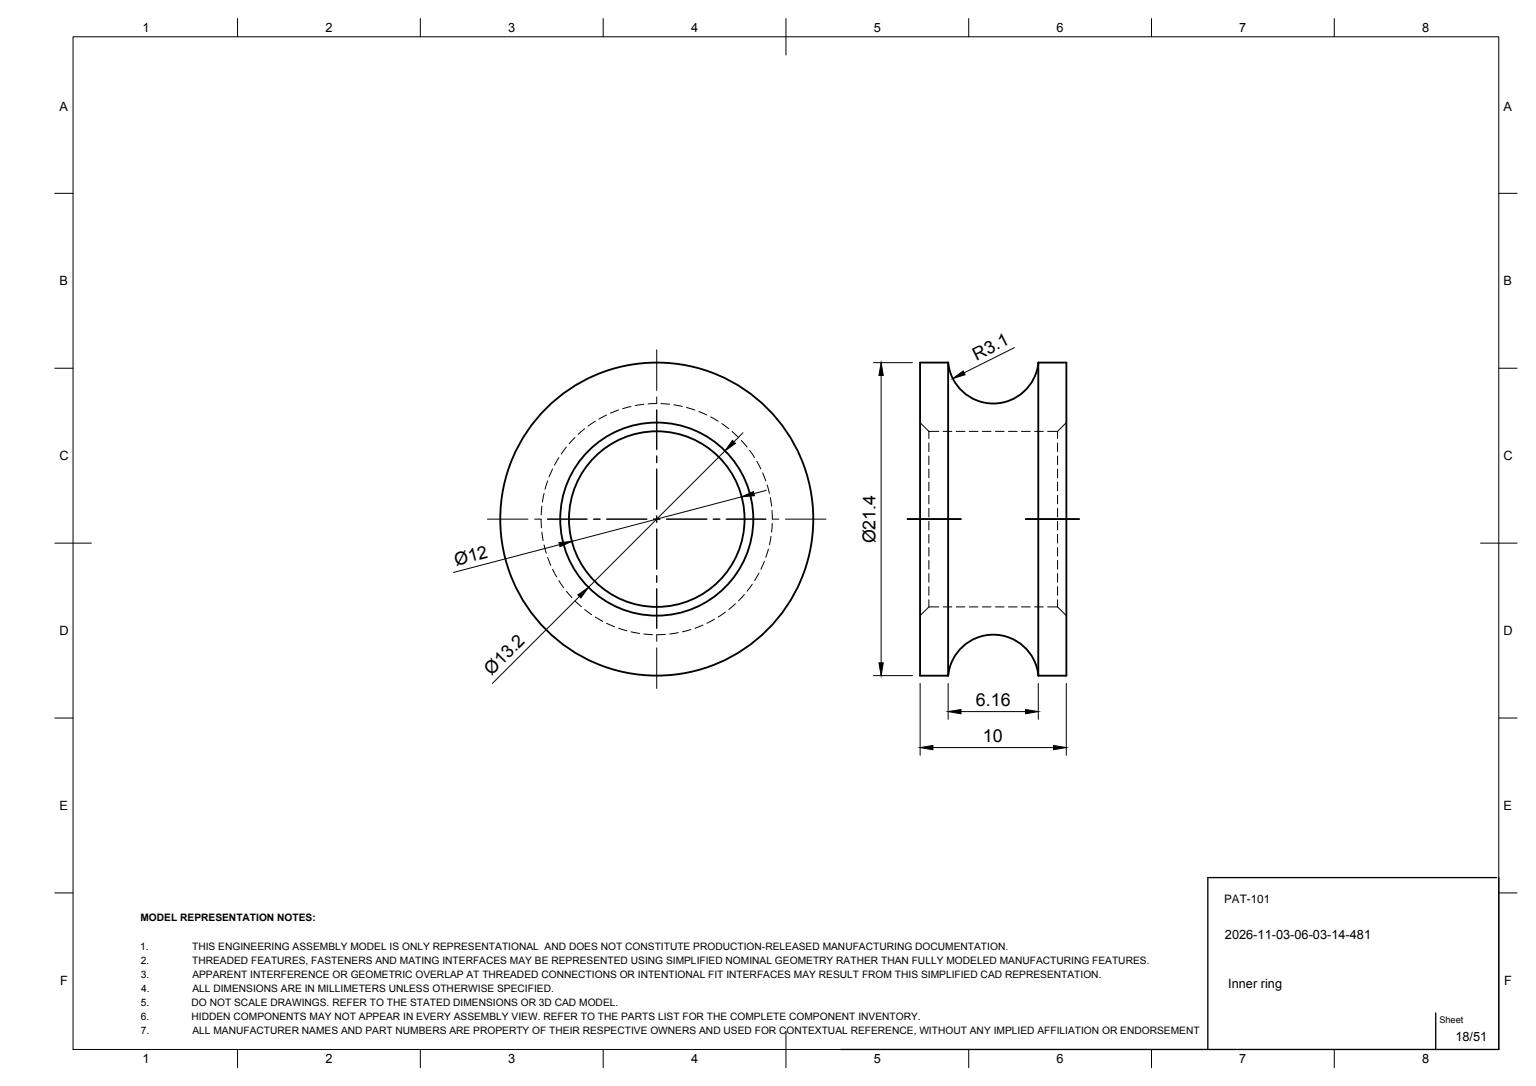
ISO-10303-21;
HEADER;
/* Generated by software containing ST-Developer
 * from STEP Tools, Inc. (www.steptools.com) 
 */

FILE_DESCRIPTION(
/* description */ ('Spur gear reduction stage 2-1 on bearing plates'),
/* implementation_level */ '2;1');

FILE_NAME(
/* name */ 'Inner ring.step',
/* time_stamp */ '2026-10-28T03:22:07-07:00',
/* author */ (''),
/* organization */ (''),
/* preprocessor_version */ 'ST-DEVELOPER v20.2',
/* originating_system */ 'Autodesk Translation Framework v15.17.0.0',
/* authorisation */ '');

FILE_SCHEMA (('AUTOMOTIVE_DESIGN { 1 0 10303 214 3 1 1 }'));
ENDSEC;

DATA;
#10=MECHANICAL_DESIGN_GEOMETRIC_PRESENTATION_REPRESENTATION('',(#960),#53909);
#825=TOROIDAL_SURFACE('',#12155,1.1,0.309556);
#840=CONICAL_SURFACE('',#12166,0.63,0.785398163397448);
#841=CONICAL_SURFACE('',#12173,0.63,0.785398163397448);
#874=SHAPE_REPRESENTATION_RELATIONSHIP('SRR','None',#54102,#917);
#917=ADVANCED_BREP_SHAPE_REPRESENTATION('',(#1016),#53876);
#960=STYLED_ITEM('',(#54397),#1016);
#1016=MANIFOLD_SOLID_BREP('Body1',#11286);
#1178=FACE_BOUND('',#2438,.T.);
#1179=FACE_BOUND('',#2441,.T.);
#1314=PLANE('',#12168);
#1315=PLANE('',#12171);
#1667=FACE_OUTER_BOUND('',#2433,.T.);
#1668=FACE_OUTER_BOUND('',#2434,.T.);
#1669=FACE_OUTER_BOUND('',#2435,.T.);
#1670=FACE_OUTER_BOUND('',#2436,.T.);
#1671=FACE_OUTER_BOUND('',#2437,.T.);
#1672=FACE_OUTER_BOUND('',#2439,.T.);
#1673=FACE_OUTER_BOUND('',#2440,.T.);
#1674=FACE_OUTER_BOUND('',#2442,.T.);
#2433=EDGE_LOOP('',(#8008,#8009,#8010,#8011,#8012,#8013));
#2434=EDGE_LOOP('',(#8014,#8015,#8016,#8017,#8018));
#2435=EDGE_LOOP('',(#8019,#8020,#8021,#8022));
#2436=EDGE_LOOP('',(#8023,#8024,#8025,#8026));
#2437=EDGE_LOOP('',(#8027));
#2438=EDGE_LOOP('',(#8028));
#2439=EDGE_LOOP('',(#8029,#8030,#8031,#8032,#8033));
#2440=EDGE_LOOP('',(#8034));
#2441=EDGE_LOOP('',(#8035));
#2442=EDGE_LOOP('',(#8036,#8037,#8038,#8039));
#3137=LINE('',#16712,#3778);
#3138=LINE('',#16718,#3779);
#3139=LINE('',#16722,#3780);
#3140=LINE('',#16728,#3781);
#3141=LINE('',#16733,#3782);
#3778=VECTOR('',#13854,1.070235);
#3779=VECTOR('',#13861,0.6);
#3780=VECTOR('',#13866,0.63);
#3781=VECTOR('',#13875,1.070235);
#3782=VECTOR('',#13882,0.63);
#4427=CIRCLE('',#12156,1.070235);
#4428=CIRCLE('',#12157,1.070235);
#4429=CIRCLE('',#12158,0.309556);
#4430=CIRCLE('',#12159,1.070235);
#4431=CIRCLE('',#12160,1.070235);
#4432=CIRCLE('',#12162,1.070235);
#4433=CIRCLE('',#12164,0.6);
#4434=CIRCLE('',#12165,0.6);
#4435=CIRCLE('',#12167,0.66);
#4436=CIRCLE('',#12170,1.070235);
#4437=CIRCLE('',#12172,0.66);
#5000=VERTEX_POINT('',#16701);
#5001=VERTEX_POINT('',#16702);
#5002=VERTEX_POINT('',#16705);
#5003=VERTEX_POINT('',#16707);
#5004=VERTEX_POINT('',#16711);
#5005=VERTEX_POINT('',#16715);
#5006=VERTEX_POINT('',#16717);
#5007=VERTEX_POINT('',#16721);
#5008=VERTEX_POINT('',#16726);
#5009=VERTEX_POINT('',#16730);
#6146=EDGE_CURVE('',#5000,#5001,#4427,.T.);
#6147=EDGE_CURVE('',#5001,#5000,#4428,.T.);
#6148=EDGE_CURVE('',#5001,#5002,#4429,.T.);
#6149=EDGE_CURVE('',#5003,#5002,#4430,.T.);
#6150=EDGE_CURVE('',#5002,#5003,#4431,.T.);
#6151=EDGE_CURVE('',#5003,#5004,#3137,.T.);
#6152=EDGE_CURVE('',#5004,#5004,#4432,.T.);
#6153=EDGE_CURVE('',#5005,#5005,#4433,.T.);
#6154=EDGE_CURVE('',#5005,#5006,#3138,.T.);
#6155=EDGE_CURVE('',#5006,#5006,#4434,.T.);
#6156=EDGE_CURVE('',#5006,#5007,#3139,.T.);
#6157=EDGE_CURVE('',#5007,#5007,#4435,.T.);
#6158=EDGE_CURVE('',#5008,#5008,#4436,.T.);
#6159=EDGE_CURVE('',#5008,#5000,#3140,.T.);
#6160=EDGE_CURVE('',#5009,#5009,#4437,.T.);
#6161=EDGE_CURVE('',#5009,#5005,#3141,.T.);
#8008=ORIENTED_EDGE('',*,*,#6146,.F.);
#8009=ORIENTED_EDGE('',*,*,#6147,.F.);
#8010=ORIENTED_EDGE('',*,*,#6148,.T.);
#8011=ORIENTED_EDGE('',*,*,#6149,.F.);
#8012=ORIENTED_EDGE('',*,*,#6150,.F.);
#8013=ORIENTED_EDGE('',*,*,#6148,.F.);
#8014=ORIENTED_EDGE('',*,*,#6149,.T.);
#8015=ORIENTED_EDGE('',*,*,#6150,.T.);
#8016=ORIENTED_EDGE('',*,*,#6151,.T.);
#8017=ORIENTED_EDGE('',*,*,#6152,.T.);
#8018=ORIENTED_EDGE('',*,*,#6151,.F.);
#8019=ORIENTED_EDGE('',*,*,#6153,.T.);
#8020=ORIENTED_EDGE('',*,*,#6154,.T.);
#8021=ORIENTED_EDGE('',*,*,#6155,.F.);
#8022=ORIENTED_EDGE('',*,*,#6154,.F.);
#8023=ORIENTED_EDGE('',*,*,#6155,.T.);
#8024=ORIENTED_EDGE('',*,*,#6156,.T.);
#8025=ORIENTED_EDGE('',*,*,#6157,.F.);
#8026=ORIENTED_EDGE('',*,*,#6156,.F.);
#8027=ORIENTED_EDGE('',*,*,#6152,.F.);
#8028=ORIENTED_EDGE('',*,*,#6157,.T.);
#8029=ORIENTED_EDGE('',*,*,#6158,.F.);
#8030=ORIENTED_EDGE('',*,*,#6159,.T.);
#8031=ORIENTED_EDGE('',*,*,#6146,.T.);
#8032=ORIENTED_EDGE('',*,*,#6147,.T.);
#8033=ORIENTED_EDGE('',*,*,#6159,.F.);
#8034=ORIENTED_EDGE('',*,*,#6158,.T.);
#8035=ORIENTED_EDGE('',*,*,#6160,.F.);
#8036=ORIENTED_EDGE('',*,*,#6160,.T.);
#8037=ORIENTED_EDGE('',*,*,#6161,.T.);
#8038=ORIENTED_EDGE('',*,*,#6153,.F.);
#8039=ORIENTED_EDGE('',*,*,#6161,.F.);
#10500=CYLINDRICAL_SURFACE('',#12161,1.070235);
#10501=CYLINDRICAL_SURFACE('',#12163,0.6);
#10502=CYLINDRICAL_SURFACE('',#12169,1.070235);
#10787=ADVANCED_FACE('',(#1667),#825,.F.);
#10788=ADVANCED_FACE('',(#1668),#10500,.T.);
#10789=ADVANCED_FACE('',(#1669),#10501,.F.);
#10790=ADVANCED_FACE('',(#1670),#840,.F.);
#10791=ADVANCED_FACE('',(#1671,#1178),#1314,.T.);
#10792=ADVANCED_FACE('',(#1672),#10502,.T.);
#10793=ADVANCED_FACE('',(#1673,#1179),#1315,.T.);
#10794=ADVANCED_FACE('',(#1674),#841,.F.);
#11286=CLOSED_SHELL('',(#10787,#10788,#10789,#10790,#10791,#10792,#10793,
#10794));
#12154=AXIS2_PLACEMENT_3D('',#16699,#13838,#13839);
#12155=AXIS2_PLACEMENT_3D('',#16700,#13840,#13841);
#12156=AXIS2_PLACEMENT_3D('',#16703,#13842,#13843);
#12157=AXIS2_PLACEMENT_3D('',#16704,#13844,#13845);
#12158=AXIS2_PLACEMENT_3D('',#16706,#13846,#13847);
#12159=AXIS2_PLACEMENT_3D('',#16708,#13848,#13849);
#12160=AXIS2_PLACEMENT_3D('',#16709,#13850,#13851);
#12161=AXIS2_PLACEMENT_3D('',#16710,#13852,#13853);
#12162=AXIS2_PLACEMENT_3D('',#16713,#13855,#13856);
#12163=AXIS2_PLACEMENT_3D('',#16714,#13857,#13858);
#12164=AXIS2_PLACEMENT_3D('',#16716,#13859,#13860);
#12165=AXIS2_PLACEMENT_3D('',#16719,#13862,#13863);
#12166=AXIS2_PLACEMENT_3D('',#16720,#13864,#13865);
#12167=AXIS2_PLACEMENT_3D('',#16723,#13867,#13868);
#12168=AXIS2_PLACEMENT_3D('',#16724,#13869,#13870);
#12169=AXIS2_PLACEMENT_3D('',#16725,#13871,#13872);
#12170=AXIS2_PLACEMENT_3D('',#16727,#13873,#13874);
#12171=AXIS2_PLACEMENT_3D('',#16729,#13876,#13877);
#12172=AXIS2_PLACEMENT_3D('',#16731,#13878,#13879);
#12173=AXIS2_PLACEMENT_3D('',#16732,#13880,#13881);
#13838=DIRECTION('axis',(0.,0.,1.));
#13839=DIRECTION('refdir',(1.,0.,0.));
#13840=DIRECTION('center_axis',(0.,-1.,0.));
#13841=DIRECTION('ref_axis',(0.,0.,-1.));
#13842=DIRECTION('center_axis',(0.,-1.,0.));
#13843=DIRECTION('ref_axis',(1.,0.,0.));
#13844=DIRECTION('center_axis',(0.,-1.,0.));
#13845=DIRECTION('ref_axis',(1.,0.,0.));
#13846=DIRECTION('center_axis',(1.,0.,1.22464679914735E-16));
#13847=DIRECTION('ref_axis',(-1.22464679914735E-16,0.,1.));
#13848=DIRECTION('center_axis',(0.,1.,0.));
#13849=DIRECTION('ref_axis',(1.,0.,0.));
#13850=DIRECTION('center_axis',(0.,1.,0.));
#13851=DIRECTION('ref_axis',(1.,0.,0.));
#13852=DIRECTION('center_axis',(0.,-1.,0.));
#13853=DIRECTION('ref_axis',(1.,0.,0.));
#13854=DIRECTION('',(0.,1.,0.));
#13855=DIRECTION('center_axis',(0.,-1.,0.));
#13856=DIRECTION('ref_axis',(1.,0.,0.));
#13857=DIRECTION('center_axis',(0.,-1.,0.));
#13858=DIRECTION('ref_axis',(1.,0.,0.));
#13859=DIRECTION('center_axis',(0.,-1.,0.));
#13860=DIRECTION('ref_axis',(1.,0.,0.));
#13861=DIRECTION('',(0.,1.,0.));
#13862=DIRECTION('center_axis',(0.,-1.,0.));
#13863=DIRECTION('ref_axis',(1.,0.,0.));
#13864=DIRECTION('center_axis',(0.,1.,0.));
#13865=DIRECTION('ref_axis',(1.,0.,0.));
#13866=DIRECTION('',(-0.707106781186548,0.707106781186547,-8.65956056235493E-17));
#13867=DIRECTION('center_axis',(0.,-1.,0.));
#13868=DIRECTION('ref_axis',(1.,0.,0.));
#13869=DIRECTION('center_axis',(0.,1.,0.));
#13870=DIRECTION('ref_axis',(0.,0.,1.));
#13871=DIRECTION('center_axis',(0.,-1.,0.));
#13872=DIRECTION('ref_axis',(1.,0.,0.));
#13873=DIRECTION('center_axis',(0.,-1.,0.));
#13874=DIRECTION('ref_axis',(1.,0.,0.));
#13875=DIRECTION('',(0.,1.,0.));
#13876=DIRECTION('center_axis',(0.,-1.,0.));
#13877=DIRECTION('ref_axis',(0.,0.,-1.));
#13878=DIRECTION('center_axis',(0.,-1.,0.));
#13879=DIRECTION('ref_axis',(1.,0.,0.));
#13880=DIRECTION('center_axis',(0.,-1.,0.));
#13881=DIRECTION('ref_axis',(1.,0.,0.));
#13882=DIRECTION('',(0.707106781186548,0.707106781186547,8.65956056235493E-17));
#16699=CARTESIAN_POINT('',(0.,0.,0.));
#16700=CARTESIAN_POINT('Origin',(0.,0.,0.));
#16701=CARTESIAN_POINT('',(-1.070235,-0.308121667383195,-1.31065986708547E-16));
#16702=CARTESIAN_POINT('',(-1.31065986708547E-16,-0.308121667383195,1.070235));
#16703=CARTESIAN_POINT('Origin',(0.,-0.308121667383195,0.));
#16704=CARTESIAN_POINT('Origin',(0.,-0.308121667383195,0.));
#16705=CARTESIAN_POINT('',(-1.31065986708547E-16,0.308121667383195,1.070235));
#16706=CARTESIAN_POINT('Origin',(-1.34711147906209E-16,0.,1.1));
#16707=CARTESIAN_POINT('',(-1.070235,0.308121667383195,1.31065986708547E-16));
#16708=CARTESIAN_POINT('Origin',(0.,0.308121667383195,0.));
#16709=CARTESIAN_POINT('Origin',(0.,0.308121667383195,0.));
#16710=CARTESIAN_POINT('Origin',(0.,0.,0.));
#16711=CARTESIAN_POINT('',(-1.070235,0.5,-1.31065986708547E-16));
#16712=CARTESIAN_POINT('',(-1.070235,0.,-1.31065986708547E-16));
#16713=CARTESIAN_POINT('Origin',(0.,0.5,0.));
#16714=CARTESIAN_POINT('Origin',(0.,0.,0.));
#16715=CARTESIAN_POINT('',(-0.6,-0.44,-7.34788079488412E-17));
#16716=CARTESIAN_POINT('Origin',(0.,-0.44,0.));
#16717=CARTESIAN_POINT('',(-0.6,0.44,-7.34788079488412E-17));
#16718=CARTESIAN_POINT('',(-0.6,0.,-7.34788079488412E-17));
#16719=CARTESIAN_POINT('Origin',(0.,0.44,0.));
#16720=CARTESIAN_POINT('Origin',(0.,0.47,0.));
#16721=CARTESIAN_POINT('',(-0.66,0.5,-8.08266887437253E-17));
#16722=CARTESIAN_POINT('',(-0.63,0.47,-7.71527483462832E-17));
#16723=CARTESIAN_POINT('Origin',(0.,0.5,0.));
#16724=CARTESIAN_POINT('Origin',(1.070235,0.5,0.));
#16725=CARTESIAN_POINT('Origin',(0.,0.,0.));
#16726=CARTESIAN_POINT('',(-1.070235,-0.5,-1.31065986708547E-16));
#16727=CARTESIAN_POINT('Origin',(0.,-0.5,0.));
#16728=CARTESIAN_POINT('',(-1.070235,0.,-1.31065986708547E-16));
#16729=CARTESIAN_POINT('Origin',(0.66,-0.5,0.));
#16730=CARTESIAN_POINT('',(-0.66,-0.5,-8.08266887437253E-17));
#16731=CARTESIAN_POINT('Origin',(0.,-0.5,0.));
#16732=CARTESIAN_POINT('Origin',(0.,-0.47,0.));
#16733=CARTESIAN_POINT('',(-0.63,-0.47,-7.71527483462832E-17));
#53826=UNCERTAINTY_MEASURE_WITH_UNIT(LENGTH_MEASURE(0.001),#53910,
'DISTANCE_ACCURACY_VALUE',
'Maximum model space distance between geometric entities at asserted c
onnectivities');
#53859=UNCERTAINTY_MEASURE_WITH_UNIT(LENGTH_MEASURE(0.001),#53910,
'DISTANCE_ACCURACY_VALUE',
'Maximum model space distance between geometric entities at asserted c
onnectivities');
#53876=(
GEOMETRIC_REPRESENTATION_CONTEXT(3)
GLOBAL_UNCERTAINTY_ASSIGNED_CONTEXT((#53826))
GLOBAL_UNIT_ASSIGNED_CONTEXT((#53910,#53912,#53913))
REPRESENTATION_CONTEXT('','3D')
);
#53909=(
GEOMETRIC_REPRESENTATION_CONTEXT(3)
GLOBAL_UNCERTAINTY_ASSIGNED_CONTEXT((#53859))
GLOBAL_UNIT_ASSIGNED_CONTEXT((#53910,#53912,#53913))
REPRESENTATION_CONTEXT('','3D')
);
#53910=(
LENGTH_UNIT()
NAMED_UNIT(*)
SI_UNIT(.CENTI.,.METRE.)
);
#53912=(
NAMED_UNIT(*)
PLANE_ANGLE_UNIT()
SI_UNIT($,.RADIAN.)
);
#53913=(
NAMED_UNIT(*)
SI_UNIT($,.STERADIAN.)
SOLID_ANGLE_UNIT()
);
#53930=SHAPE_DEFINITION_REPRESENTATION(#53979,#54102);
#53979=PRODUCT_DEFINITION_SHAPE('',$,#54152);
#54102=SHAPE_REPRESENTATION('',(#12154),#53876);
#54135=PRODUCT_DEFINITION_CONTEXT('part definition',#54284,'design');
#54152=PRODUCT_DEFINITION('Inner ring','Inner ring',#54201,#54135);
#54201=PRODUCT_DEFINITION_FORMATION('',$,#54302);
#54284=APPLICATION_CONTEXT(
'Core Data for Automotive Mechanical Design Process');
#54285=PRODUCT_CONTEXT('part definition',#54284,'mechanical');
#54302=PRODUCT('Inner ring','Inner ring','Inner ring',(#54285));
#54391=COLOUR_RGB('Grey',0.48,0.52,0.57);
#54392=FILL_AREA_STYLE_COLOUR('',#54391);
#54393=FILL_AREA_STYLE('',(#54392));
#54394=SURFACE_STYLE_FILL_AREA(#54393);
#54395=SURFACE_SIDE_STYLE('',(#54394));
#54396=SURFACE_STYLE_USAGE(.BOTH.,#54395);
#54397=PRESENTATION_STYLE_ASSIGNMENT((#54396));
ENDSEC;
END-ISO-10303-21;
